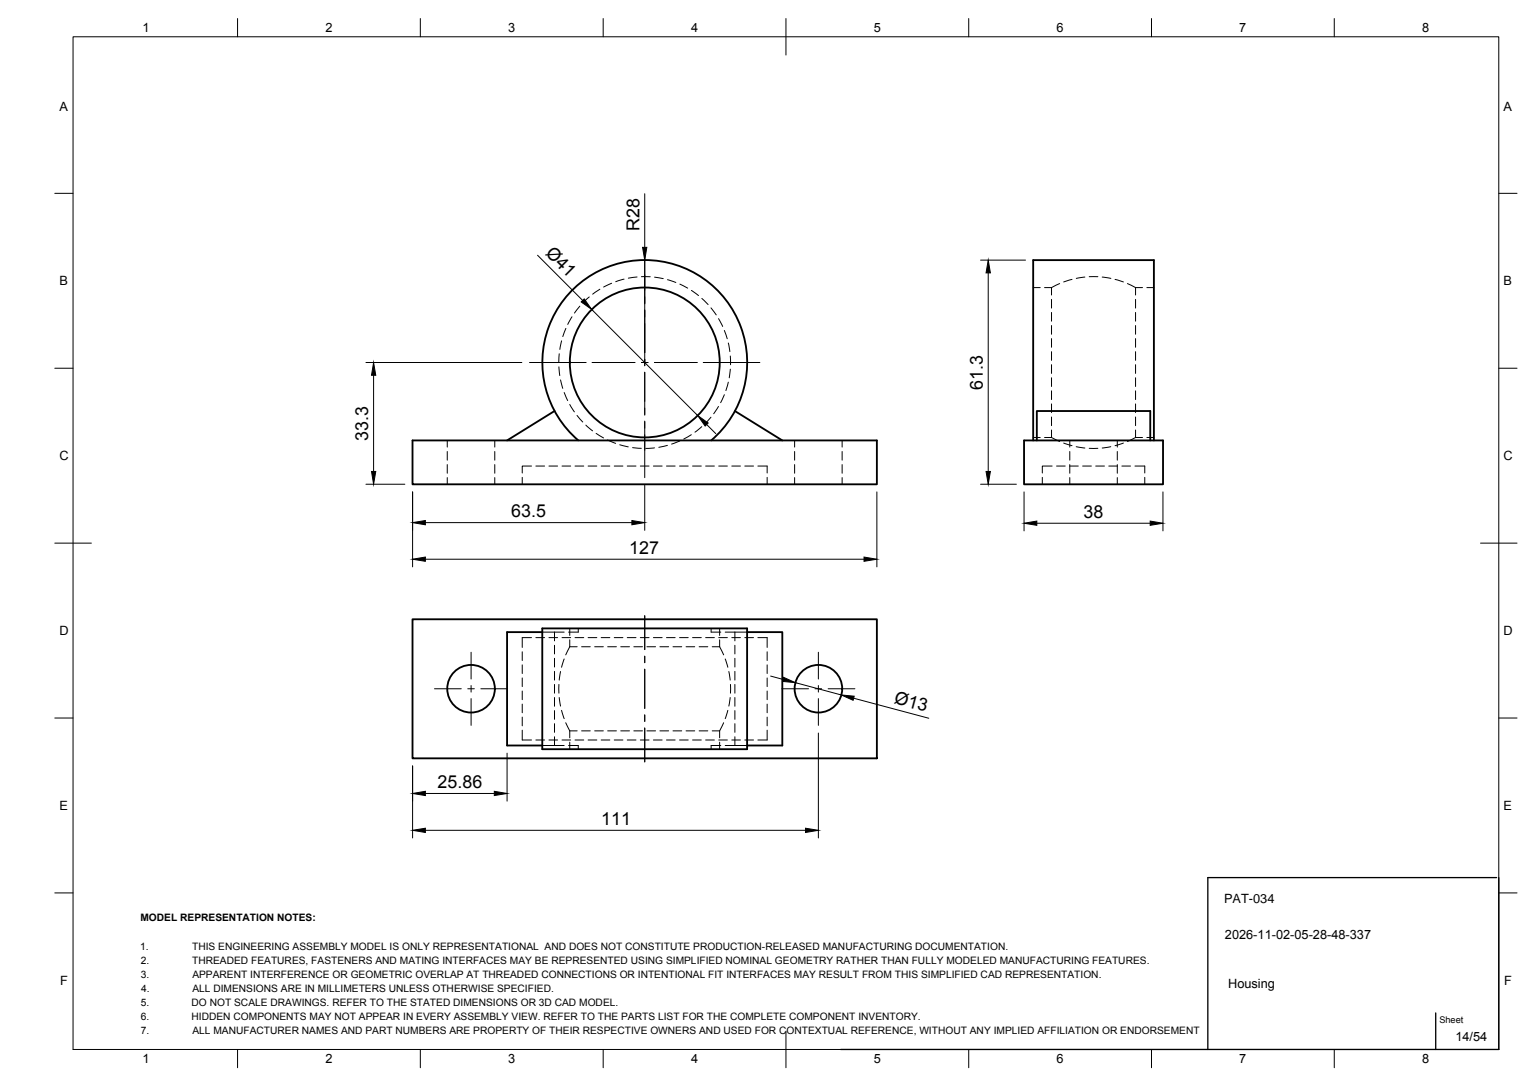
ISO-10303-21;
HEADER;
/* Generated by software containing ST-Developer
 * from STEP Tools, Inc. (www.steptools.com) 
 */

FILE_DESCRIPTION(
/* description */ ('Fatigue rig crank-slider'),
/* implementation_level */ '2;1');

FILE_NAME(
/* name */ 'Housing.step',
/* time_stamp */ '2026-10-28T03:24:50-07:00',
/* author */ (''),
/* organization */ (''),
/* preprocessor_version */ 'ST-DEVELOPER v20.2',
/* originating_system */ 'Autodesk Translation Framework v15.17.0.0',
/* authorisation */ '');

FILE_SCHEMA (('AUTOMOTIVE_DESIGN { 1 0 10303 214 3 1 1 }'));
ENDSEC;

DATA;
#10=MECHANICAL_DESIGN_GEOMETRIC_PRESENTATION_REPRESENTATION('',(#597),#16911);
#469=SPHERICAL_SURFACE('',#9733,2.35);
#497=SHAPE_REPRESENTATION_RELATIONSHIP('SRR','None',#17137,#547);
#547=ADVANCED_BREP_SHAPE_REPRESENTATION('',(#656),#16866);
#597=STYLED_ITEM('',(#17466),#656);
#656=MANIFOLD_SOLID_BREP('Body1',#8888);
#776=FACE_BOUND('',#1935,.T.);
#777=FACE_BOUND('',#1936,.T.);
#778=FACE_BOUND('',#1944,.T.);
#779=FACE_BOUND('',#1945,.T.);
#780=FACE_BOUND('',#1946,.T.);
#781=FACE_BOUND('',#1949,.T.);
#782=FACE_BOUND('',#1951,.T.);
#783=FACE_BOUND('',#1964,.T.);
#784=FACE_BOUND('',#1965,.T.);
#785=FACE_BOUND('',#1966,.T.);
#961=PLANE('',#9735);
#962=PLANE('',#9737);
#963=PLANE('',#9739);
#964=PLANE('',#9741);
#965=PLANE('',#9742);
#966=PLANE('',#9744);
#967=PLANE('',#9745);
#968=PLANE('',#9751);
#969=PLANE('',#9752);
#970=PLANE('',#9753);
#971=PLANE('',#9754);
#972=PLANE('',#9755);
#973=PLANE('',#9756);
#974=PLANE('',#9757);
#975=PLANE('',#9762);
#976=PLANE('',#9763);
#977=PLANE('',#9764);
#978=PLANE('',#9765);
#979=PLANE('',#9766);
#1333=FACE_OUTER_BOUND('',#1932,.T.);
#1334=FACE_OUTER_BOUND('',#1933,.T.);
#1335=FACE_OUTER_BOUND('',#1934,.T.);
#1336=FACE_OUTER_BOUND('',#1937,.T.);
#1337=FACE_OUTER_BOUND('',#1938,.T.);
#1338=FACE_OUTER_BOUND('',#1939,.T.);
#1339=FACE_OUTER_BOUND('',#1940,.T.);
#1340=FACE_OUTER_BOUND('',#1941,.T.);
#1341=FACE_OUTER_BOUND('',#1942,.T.);
#1342=FACE_OUTER_BOUND('',#1943,.T.);
#1343=FACE_OUTER_BOUND('',#1947,.T.);
#1344=FACE_OUTER_BOUND('',#1948,.T.);
#1345=FACE_OUTER_BOUND('',#1950,.T.);
#1346=FACE_OUTER_BOUND('',#1952,.T.);
#1347=FACE_OUTER_BOUND('',#1953,.T.);
#1348=FACE_OUTER_BOUND('',#1954,.T.);
#1349=FACE_OUTER_BOUND('',#1955,.T.);
#1350=FACE_OUTER_BOUND('',#1956,.T.);
#1351=FACE_OUTER_BOUND('',#1957,.T.);
#1352=FACE_OUTER_BOUND('',#1958,.T.);
#1353=FACE_OUTER_BOUND('',#1959,.T.);
#1354=FACE_OUTER_BOUND('',#1960,.T.);
#1355=FACE_OUTER_BOUND('',#1961,.T.);
#1356=FACE_OUTER_BOUND('',#1962,.T.);
#1357=FACE_OUTER_BOUND('',#1963,.T.);
#1932=EDGE_LOOP('',(#6452,#6453,#6454,#6455));
#1933=EDGE_LOOP('',(#6456,#6457,#6458,#6459));
#1934=EDGE_LOOP('',(#6460,#6461));
#1935=EDGE_LOOP('',(#6462));
#1936=EDGE_LOOP('',(#6463));
#1937=EDGE_LOOP('',(#6464,#6465,#6466));
#1938=EDGE_LOOP('',(#6467,#6468,#6469));
#1939=EDGE_LOOP('',(#6470,#6471,#6472));
#1940=EDGE_LOOP('',(#6473,#6474,#6475,#6476));
#1941=EDGE_LOOP('',(#6477,#6478,#6479));
#1942=EDGE_LOOP('',(#6480,#6481,#6482,#6483));
#1943=EDGE_LOOP('',(#6484,#6485,#6486,#6487));
#1944=EDGE_LOOP('',(#6488));
#1945=EDGE_LOOP('',(#6489));
#1946=EDGE_LOOP('',(#6490,#6491,#6492,#6493,#6494,#6495,#6496,#6497,#6498,
#6499,#6500,#6501));
#1947=EDGE_LOOP('',(#6502,#6503,#6504,#6505,#6506,#6507,#6508,#6509,#6510,
#6511,#6512,#6513));
#1948=EDGE_LOOP('',(#6514,#6515));
#1949=EDGE_LOOP('',(#6516));
#1950=EDGE_LOOP('',(#6517,#6518));
#1951=EDGE_LOOP('',(#6519));
#1952=EDGE_LOOP('',(#6520,#6521,#6522,#6523));
#1953=EDGE_LOOP('',(#6524,#6525,#6526,#6527));
#1954=EDGE_LOOP('',(#6528,#6529,#6530,#6531));
#1955=EDGE_LOOP('',(#6532,#6533,#6534,#6535));
#1956=EDGE_LOOP('',(#6536,#6537,#6538,#6539));
#1957=EDGE_LOOP('',(#6540,#6541,#6542,#6543));
#1958=EDGE_LOOP('',(#6544,#6545,#6546,#6547));
#1959=EDGE_LOOP('',(#6548,#6549,#6550,#6551));
#1960=EDGE_LOOP('',(#6552,#6553,#6554,#6555));
#1961=EDGE_LOOP('',(#6556,#6557,#6558,#6559));
#1962=EDGE_LOOP('',(#6560,#6561,#6562,#6563));
#1963=EDGE_LOOP('',(#6564,#6565,#6566,#6567));
#1964=EDGE_LOOP('',(#6568,#6569,#6570,#6571));
#1965=EDGE_LOOP('',(#6572));
#1966=EDGE_LOOP('',(#6573));
#2584=LINE('',#13872,#3230);
#2585=LINE('',#13878,#3231);
#2586=LINE('',#13887,#3232);
#2587=LINE('',#13889,#3233);
#2588=LINE('',#13894,#3234);
#2589=LINE('',#13897,#3235);
#2590=LINE('',#13901,#3236);
#2591=LINE('',#13904,#3237);
#2592=LINE('',#13906,#3238);
#2593=LINE('',#13907,#3239);
#2594=LINE('',#13911,#3240);
#2595=LINE('',#13913,#3241);
#2596=LINE('',#13916,#3242);
#2597=LINE('',#13917,#3243);
#2598=LINE('',#13921,#3244);
#2599=LINE('',#13923,#3245);
#2600=LINE('',#13925,#3246);
#2601=LINE('',#13926,#3247);
#2602=LINE('',#13932,#3248);
#2603=LINE('',#13934,#3249);
#2604=LINE('',#13935,#3250);
#2605=LINE('',#13937,#3251);
#2606=LINE('',#13939,#3252);
#2607=LINE('',#13940,#3253);
#2608=LINE('',#13949,#3254);
#2609=LINE('',#13951,#3255);
#2610=LINE('',#13953,#3256);
#2611=LINE('',#13954,#3257);
#2612=LINE('',#13957,#3258);
#2613=LINE('',#13959,#3259);
#2614=LINE('',#13960,#3260);
#2615=LINE('',#13963,#3261);
#2616=LINE('',#13965,#3262);
#2617=LINE('',#13966,#3263);
#2618=LINE('',#13968,#3264);
#2619=LINE('',#13969,#3265);
#2620=LINE('',#13974,#3266);
#2621=LINE('',#13978,#3267);
#2622=LINE('',#13982,#3268);
#2623=LINE('',#13983,#3269);
#2624=LINE('',#13984,#3270);
#2625=LINE('',#13987,#3271);
#2626=LINE('',#13988,#3272);
#2627=LINE('',#13991,#3273);
#2628=LINE('',#13992,#3274);
#2629=LINE('',#13994,#3275);
#3230=VECTOR('',#11162,2.05);
#3231=VECTOR('',#11169,2.05);
#3232=VECTOR('',#11178,1.);
#3233=VECTOR('',#11179,1.);
#3234=VECTOR('',#11184,1.);
#3235=VECTOR('',#11187,1.);
#3236=VECTOR('',#11190,1.);
#3237=VECTOR('',#11193,1.);
#3238=VECTOR('',#11196,1.);
#3239=VECTOR('',#11197,1.);
#3240=VECTOR('',#11200,1.);
#3241=VECTOR('',#11201,1.);
#3242=VECTOR('',#11206,1.);
#3243=VECTOR('',#11207,1.);
#3244=VECTOR('',#11210,1.);
#3245=VECTOR('',#11211,1.);
#3246=VECTOR('',#11212,1.);
#3247=VECTOR('',#11213,1.);
#3248=VECTOR('',#11218,1.);
#3249=VECTOR('',#11219,1.);
#3250=VECTOR('',#11220,1.);
#3251=VECTOR('',#11221,1.);
#3252=VECTOR('',#11222,1.);
#3253=VECTOR('',#11223,1.);
#3254=VECTOR('',#11236,1.);
#3255=VECTOR('',#11237,1.);
#3256=VECTOR('',#11238,1.);
#3257=VECTOR('',#11239,1.);
#3258=VECTOR('',#11242,1.);
#3259=VECTOR('',#11243,1.);
#3260=VECTOR('',#11244,1.);
#3261=VECTOR('',#11247,1.);
#3262=VECTOR('',#11248,1.);
#3263=VECTOR('',#11249,1.);
#3264=VECTOR('',#11252,1.);
#3265=VECTOR('',#11253,1.);
#3266=VECTOR('',#11260,0.65);
#3267=VECTOR('',#11265,0.65);
#3268=VECTOR('',#11268,1.);
#3269=VECTOR('',#11269,1.);
#3270=VECTOR('',#11270,1.);
#3271=VECTOR('',#11273,1.);
#3272=VECTOR('',#11274,1.);
#3273=VECTOR('',#11277,1.);
#3274=VECTOR('',#11278,1.);
#3275=VECTOR('',#11281,1.);
#3856=CIRCLE('',#9728,2.05);
#3857=CIRCLE('',#9729,2.05);
#3858=CIRCLE('',#9731,2.05);
#3859=CIRCLE('',#9732,2.05);
#3860=CIRCLE('',#9734,2.35);
#3861=CIRCLE('',#9736,2.8);
#3862=CIRCLE('',#9738,2.8);
#3863=CIRCLE('',#9740,2.8);
#3864=CIRCLE('',#9743,2.8);
#3865=CIRCLE('',#9746,0.65);
#3866=CIRCLE('',#9747,0.65);
#3867=CIRCLE('',#9749,2.8);
#3868=CIRCLE('',#9750,2.8);
#3869=CIRCLE('',#9759,0.65);
#3870=CIRCLE('',#9761,0.65);
#4304=VERTEX_POINT('',#13869);
#4305=VERTEX_POINT('',#13871);
#4306=VERTEX_POINT('',#13875);
#4307=VERTEX_POINT('',#13877);
#4308=VERTEX_POINT('',#13881);
#4309=VERTEX_POINT('',#13882);
#4310=VERTEX_POINT('',#13885);
#4311=VERTEX_POINT('',#13886);
#4312=VERTEX_POINT('',#13888);
#4313=VERTEX_POINT('',#13892);
#4314=VERTEX_POINT('',#13893);
#4315=VERTEX_POINT('',#13895);
#4316=VERTEX_POINT('',#13899);
#4317=VERTEX_POINT('',#13900);
#4318=VERTEX_POINT('',#13902);
#4319=VERTEX_POINT('',#13909);
#4320=VERTEX_POINT('',#13910);
#4321=VERTEX_POINT('',#13912);
#4322=VERTEX_POINT('',#13919);
#4323=VERTEX_POINT('',#13920);
#4324=VERTEX_POINT('',#13922);
#4325=VERTEX_POINT('',#13924);
#4326=VERTEX_POINT('',#13927);
#4327=VERTEX_POINT('',#13929);
#4328=VERTEX_POINT('',#13931);
#4329=VERTEX_POINT('',#13933);
#4330=VERTEX_POINT('',#13936);
#4331=VERTEX_POINT('',#13938);
#4332=VERTEX_POINT('',#13947);
#4333=VERTEX_POINT('',#13948);
#4334=VERTEX_POINT('',#13950);
#4335=VERTEX_POINT('',#13952);
#4336=VERTEX_POINT('',#13956);
#4337=VERTEX_POINT('',#13958);
#4338=VERTEX_POINT('',#13962);
#4339=VERTEX_POINT('',#13964);
#4340=VERTEX_POINT('',#13972);
#4341=VERTEX_POINT('',#13976);
#4342=VERTEX_POINT('',#13980);
#4343=VERTEX_POINT('',#13981);
#4344=VERTEX_POINT('',#13986);
#4345=VERTEX_POINT('',#13990);
#5124=EDGE_CURVE('',#4304,#4304,#3856,.T.);
#5125=EDGE_CURVE('',#4304,#4305,#2584,.T.);
#5126=EDGE_CURVE('',#4305,#4305,#3857,.T.);
#5127=EDGE_CURVE('',#4306,#4306,#3858,.T.);
#5128=EDGE_CURVE('',#4306,#4307,#2585,.T.);
#5129=EDGE_CURVE('',#4307,#4307,#3859,.T.);
#5130=EDGE_CURVE('',#4308,#4309,#3860,.T.);
#5131=EDGE_CURVE('',#4310,#4311,#2586,.T.);
#5132=EDGE_CURVE('',#4310,#4312,#2587,.T.);
#5133=EDGE_CURVE('',#4311,#4312,#3861,.T.);
#5134=EDGE_CURVE('',#4313,#4314,#2588,.T.);
#5135=EDGE_CURVE('',#4315,#4313,#3862,.T.);
#5136=EDGE_CURVE('',#4315,#4314,#2589,.T.);
#5137=EDGE_CURVE('',#4316,#4317,#2590,.T.);
#5138=EDGE_CURVE('',#4318,#4316,#3863,.T.);
#5139=EDGE_CURVE('',#4318,#4317,#2591,.T.);
#5140=EDGE_CURVE('',#4317,#4310,#2592,.T.);
#5141=EDGE_CURVE('',#4312,#4318,#2593,.T.);
#5142=EDGE_CURVE('',#4319,#4320,#2594,.T.);
#5143=EDGE_CURVE('',#4319,#4321,#2595,.T.);
#5144=EDGE_CURVE('',#4320,#4321,#3864,.T.);
#5145=EDGE_CURVE('',#4314,#4319,#2596,.T.);
#5146=EDGE_CURVE('',#4321,#4315,#2597,.T.);
#5147=EDGE_CURVE('',#4322,#4323,#2598,.T.);
#5148=EDGE_CURVE('',#4323,#4324,#2599,.T.);
#5149=EDGE_CURVE('',#4324,#4325,#2600,.T.);
#5150=EDGE_CURVE('',#4325,#4322,#2601,.T.);
#5151=EDGE_CURVE('',#4326,#4326,#3865,.T.);
#5152=EDGE_CURVE('',#4327,#4327,#3866,.T.);
#5153=EDGE_CURVE('',#4320,#4328,#2602,.T.);
#5154=EDGE_CURVE('',#4328,#4329,#2603,.T.);
#5155=EDGE_CURVE('',#4329,#4316,#2604,.T.);
#5156=EDGE_CURVE('',#4311,#4330,#2605,.T.);
#5157=EDGE_CURVE('',#4330,#4331,#2606,.T.);
#5158=EDGE_CURVE('',#4331,#4313,#2607,.T.);
#5159=EDGE_CURVE('',#4330,#4331,#3867,.T.);
#5160=EDGE_CURVE('',#4328,#4329,#3868,.T.);
#5161=EDGE_CURVE('',#4332,#4333,#2608,.T.);
#5162=EDGE_CURVE('',#4332,#4334,#2609,.T.);
#5163=EDGE_CURVE('',#4334,#4335,#2610,.T.);
#5164=EDGE_CURVE('',#4333,#4335,#2611,.T.);
#5165=EDGE_CURVE('',#4336,#4332,#2612,.T.);
#5166=EDGE_CURVE('',#4336,#4337,#2613,.T.);
#5167=EDGE_CURVE('',#4337,#4334,#2614,.T.);
#5168=EDGE_CURVE('',#4338,#4336,#2615,.T.);
#5169=EDGE_CURVE('',#4338,#4339,#2616,.T.);
#5170=EDGE_CURVE('',#4339,#4337,#2617,.T.);
#5171=EDGE_CURVE('',#4333,#4338,#2618,.T.);
#5172=EDGE_CURVE('',#4335,#4339,#2619,.T.);
#5173=EDGE_CURVE('',#4340,#4340,#3869,.T.);
#5174=EDGE_CURVE('',#4340,#4327,#2620,.T.);
#5175=EDGE_CURVE('',#4341,#4341,#3870,.T.);
#5176=EDGE_CURVE('',#4341,#4326,#2621,.T.);
#5177=EDGE_CURVE('',#4342,#4343,#2622,.T.);
#5178=EDGE_CURVE('',#4343,#4322,#2623,.T.);
#5179=EDGE_CURVE('',#4342,#4325,#2624,.T.);
#5180=EDGE_CURVE('',#4344,#4342,#2625,.T.);
#5181=EDGE_CURVE('',#4344,#4324,#2626,.T.);
#5182=EDGE_CURVE('',#4345,#4344,#2627,.T.);
#5183=EDGE_CURVE('',#4345,#4323,#2628,.T.);
#5184=EDGE_CURVE('',#4343,#4345,#2629,.T.);
#6452=ORIENTED_EDGE('',*,*,#5124,.F.);
#6453=ORIENTED_EDGE('',*,*,#5125,.T.);
#6454=ORIENTED_EDGE('',*,*,#5126,.F.);
#6455=ORIENTED_EDGE('',*,*,#5125,.F.);
#6456=ORIENTED_EDGE('',*,*,#5127,.F.);
#6457=ORIENTED_EDGE('',*,*,#5128,.T.);
#6458=ORIENTED_EDGE('',*,*,#5129,.F.);
#6459=ORIENTED_EDGE('',*,*,#5128,.F.);
#6460=ORIENTED_EDGE('',*,*,#5130,.T.);
#6461=ORIENTED_EDGE('',*,*,#5130,.F.);
#6462=ORIENTED_EDGE('',*,*,#5127,.T.);
#6463=ORIENTED_EDGE('',*,*,#5126,.T.);
#6464=ORIENTED_EDGE('',*,*,#5131,.F.);
#6465=ORIENTED_EDGE('',*,*,#5132,.T.);
#6466=ORIENTED_EDGE('',*,*,#5133,.F.);
#6467=ORIENTED_EDGE('',*,*,#5134,.F.);
#6468=ORIENTED_EDGE('',*,*,#5135,.F.);
#6469=ORIENTED_EDGE('',*,*,#5136,.T.);
#6470=ORIENTED_EDGE('',*,*,#5137,.F.);
#6471=ORIENTED_EDGE('',*,*,#5138,.F.);
#6472=ORIENTED_EDGE('',*,*,#5139,.T.);
#6473=ORIENTED_EDGE('',*,*,#5140,.F.);
#6474=ORIENTED_EDGE('',*,*,#5139,.F.);
#6475=ORIENTED_EDGE('',*,*,#5141,.F.);
#6476=ORIENTED_EDGE('',*,*,#5132,.F.);
#6477=ORIENTED_EDGE('',*,*,#5142,.F.);
#6478=ORIENTED_EDGE('',*,*,#5143,.T.);
#6479=ORIENTED_EDGE('',*,*,#5144,.F.);
#6480=ORIENTED_EDGE('',*,*,#5145,.F.);
#6481=ORIENTED_EDGE('',*,*,#5136,.F.);
#6482=ORIENTED_EDGE('',*,*,#5146,.F.);
#6483=ORIENTED_EDGE('',*,*,#5143,.F.);
#6484=ORIENTED_EDGE('',*,*,#5147,.T.);
#6485=ORIENTED_EDGE('',*,*,#5148,.T.);
#6486=ORIENTED_EDGE('',*,*,#5149,.T.);
#6487=ORIENTED_EDGE('',*,*,#5150,.T.);
#6488=ORIENTED_EDGE('',*,*,#5151,.T.);
#6489=ORIENTED_EDGE('',*,*,#5152,.T.);
#6490=ORIENTED_EDGE('',*,*,#5134,.T.);
#6491=ORIENTED_EDGE('',*,*,#5145,.T.);
#6492=ORIENTED_EDGE('',*,*,#5142,.T.);
#6493=ORIENTED_EDGE('',*,*,#5153,.T.);
#6494=ORIENTED_EDGE('',*,*,#5154,.T.);
#6495=ORIENTED_EDGE('',*,*,#5155,.T.);
#6496=ORIENTED_EDGE('',*,*,#5137,.T.);
#6497=ORIENTED_EDGE('',*,*,#5140,.T.);
#6498=ORIENTED_EDGE('',*,*,#5131,.T.);
#6499=ORIENTED_EDGE('',*,*,#5156,.T.);
#6500=ORIENTED_EDGE('',*,*,#5157,.T.);
#6501=ORIENTED_EDGE('',*,*,#5158,.T.);
#6502=ORIENTED_EDGE('',*,*,#5135,.T.);
#6503=ORIENTED_EDGE('',*,*,#5158,.F.);
#6504=ORIENTED_EDGE('',*,*,#5159,.F.);
#6505=ORIENTED_EDGE('',*,*,#5156,.F.);
#6506=ORIENTED_EDGE('',*,*,#5133,.T.);
#6507=ORIENTED_EDGE('',*,*,#5141,.T.);
#6508=ORIENTED_EDGE('',*,*,#5138,.T.);
#6509=ORIENTED_EDGE('',*,*,#5155,.F.);
#6510=ORIENTED_EDGE('',*,*,#5160,.F.);
#6511=ORIENTED_EDGE('',*,*,#5153,.F.);
#6512=ORIENTED_EDGE('',*,*,#5144,.T.);
#6513=ORIENTED_EDGE('',*,*,#5146,.T.);
#6514=ORIENTED_EDGE('',*,*,#5154,.F.);
#6515=ORIENTED_EDGE('',*,*,#5160,.T.);
#6516=ORIENTED_EDGE('',*,*,#5124,.T.);
#6517=ORIENTED_EDGE('',*,*,#5157,.F.);
#6518=ORIENTED_EDGE('',*,*,#5159,.T.);
#6519=ORIENTED_EDGE('',*,*,#5129,.T.);
#6520=ORIENTED_EDGE('',*,*,#5161,.F.);
#6521=ORIENTED_EDGE('',*,*,#5162,.T.);
#6522=ORIENTED_EDGE('',*,*,#5163,.T.);
#6523=ORIENTED_EDGE('',*,*,#5164,.F.);
#6524=ORIENTED_EDGE('',*,*,#5165,.F.);
#6525=ORIENTED_EDGE('',*,*,#5166,.T.);
#6526=ORIENTED_EDGE('',*,*,#5167,.T.);
#6527=ORIENTED_EDGE('',*,*,#5162,.F.);
#6528=ORIENTED_EDGE('',*,*,#5168,.F.);
#6529=ORIENTED_EDGE('',*,*,#5169,.T.);
#6530=ORIENTED_EDGE('',*,*,#5170,.T.);
#6531=ORIENTED_EDGE('',*,*,#5166,.F.);
#6532=ORIENTED_EDGE('',*,*,#5171,.F.);
#6533=ORIENTED_EDGE('',*,*,#5164,.T.);
#6534=ORIENTED_EDGE('',*,*,#5172,.T.);
#6535=ORIENTED_EDGE('',*,*,#5169,.F.);
#6536=ORIENTED_EDGE('',*,*,#5172,.F.);
#6537=ORIENTED_EDGE('',*,*,#5163,.F.);
#6538=ORIENTED_EDGE('',*,*,#5167,.F.);
#6539=ORIENTED_EDGE('',*,*,#5170,.F.);
#6540=ORIENTED_EDGE('',*,*,#5173,.F.);
#6541=ORIENTED_EDGE('',*,*,#5174,.T.);
#6542=ORIENTED_EDGE('',*,*,#5152,.F.);
#6543=ORIENTED_EDGE('',*,*,#5174,.F.);
#6544=ORIENTED_EDGE('',*,*,#5175,.F.);
#6545=ORIENTED_EDGE('',*,*,#5176,.T.);
#6546=ORIENTED_EDGE('',*,*,#5151,.F.);
#6547=ORIENTED_EDGE('',*,*,#5176,.F.);
#6548=ORIENTED_EDGE('',*,*,#5177,.T.);
#6549=ORIENTED_EDGE('',*,*,#5178,.T.);
#6550=ORIENTED_EDGE('',*,*,#5150,.F.);
#6551=ORIENTED_EDGE('',*,*,#5179,.F.);
#6552=ORIENTED_EDGE('',*,*,#5180,.T.);
#6553=ORIENTED_EDGE('',*,*,#5179,.T.);
#6554=ORIENTED_EDGE('',*,*,#5149,.F.);
#6555=ORIENTED_EDGE('',*,*,#5181,.F.);
#6556=ORIENTED_EDGE('',*,*,#5182,.T.);
#6557=ORIENTED_EDGE('',*,*,#5181,.T.);
#6558=ORIENTED_EDGE('',*,*,#5148,.F.);
#6559=ORIENTED_EDGE('',*,*,#5183,.F.);
#6560=ORIENTED_EDGE('',*,*,#5184,.T.);
#6561=ORIENTED_EDGE('',*,*,#5183,.T.);
#6562=ORIENTED_EDGE('',*,*,#5147,.F.);
#6563=ORIENTED_EDGE('',*,*,#5178,.F.);
#6564=ORIENTED_EDGE('',*,*,#5184,.F.);
#6565=ORIENTED_EDGE('',*,*,#5177,.F.);
#6566=ORIENTED_EDGE('',*,*,#5180,.F.);
#6567=ORIENTED_EDGE('',*,*,#5182,.F.);
#6568=ORIENTED_EDGE('',*,*,#5161,.T.);
#6569=ORIENTED_EDGE('',*,*,#5171,.T.);
#6570=ORIENTED_EDGE('',*,*,#5168,.T.);
#6571=ORIENTED_EDGE('',*,*,#5165,.T.);
#6572=ORIENTED_EDGE('',*,*,#5173,.T.);
#6573=ORIENTED_EDGE('',*,*,#5175,.T.);
#8248=CYLINDRICAL_SURFACE('',#9727,2.05);
#8249=CYLINDRICAL_SURFACE('',#9730,2.05);
#8250=CYLINDRICAL_SURFACE('',#9748,2.8);
#8251=CYLINDRICAL_SURFACE('',#9758,0.65);
#8252=CYLINDRICAL_SURFACE('',#9760,0.65);
#8471=ADVANCED_FACE('',(#1333),#8248,.F.);
#8472=ADVANCED_FACE('',(#1334),#8249,.F.);
#8473=ADVANCED_FACE('',(#1335,#776,#777),#469,.F.);
#8474=ADVANCED_FACE('',(#1336),#961,.T.);
#8475=ADVANCED_FACE('',(#1337),#962,.T.);
#8476=ADVANCED_FACE('',(#1338),#963,.T.);
#8477=ADVANCED_FACE('',(#1339),#964,.T.);
#8478=ADVANCED_FACE('',(#1340),#965,.T.);
#8479=ADVANCED_FACE('',(#1341),#966,.T.);
#8480=ADVANCED_FACE('',(#1342,#778,#779,#780),#967,.T.);
#8481=ADVANCED_FACE('',(#1343),#8250,.T.);
#8482=ADVANCED_FACE('',(#1344,#781),#968,.F.);
#8483=ADVANCED_FACE('',(#1345,#782),#969,.T.);
#8484=ADVANCED_FACE('',(#1346),#970,.F.);
#8485=ADVANCED_FACE('',(#1347),#971,.F.);
#8486=ADVANCED_FACE('',(#1348),#972,.F.);
#8487=ADVANCED_FACE('',(#1349),#973,.F.);
#8488=ADVANCED_FACE('',(#1350),#974,.F.);
#8489=ADVANCED_FACE('',(#1351),#8251,.F.);
#8490=ADVANCED_FACE('',(#1352),#8252,.F.);
#8491=ADVANCED_FACE('',(#1353),#975,.T.);
#8492=ADVANCED_FACE('',(#1354),#976,.T.);
#8493=ADVANCED_FACE('',(#1355),#977,.T.);
#8494=ADVANCED_FACE('',(#1356),#978,.T.);
#8495=ADVANCED_FACE('',(#1357,#783,#784,#785),#979,.F.);
#8888=CLOSED_SHELL('',(#8471,#8472,#8473,#8474,#8475,#8476,#8477,#8478,
#8479,#8480,#8481,#8482,#8483,#8484,#8485,#8486,#8487,#8488,#8489,#8490,
#8491,#8492,#8493,#8494,#8495));
#9726=AXIS2_PLACEMENT_3D('',#13867,#11156,#11157);
#9727=AXIS2_PLACEMENT_3D('',#13868,#11158,#11159);
#9728=AXIS2_PLACEMENT_3D('',#13870,#11160,#11161);
#9729=AXIS2_PLACEMENT_3D('',#13873,#11163,#11164);
#9730=AXIS2_PLACEMENT_3D('',#13874,#11165,#11166);
#9731=AXIS2_PLACEMENT_3D('',#13876,#11167,#11168);
#9732=AXIS2_PLACEMENT_3D('',#13879,#11170,#11171);
#9733=AXIS2_PLACEMENT_3D('',#13880,#11172,#11173);
#9734=AXIS2_PLACEMENT_3D('',#13883,#11174,#11175);
#9735=AXIS2_PLACEMENT_3D('',#13884,#11176,#11177);
#9736=AXIS2_PLACEMENT_3D('',#13890,#11180,#11181);
#9737=AXIS2_PLACEMENT_3D('',#13891,#11182,#11183);
#9738=AXIS2_PLACEMENT_3D('',#13896,#11185,#11186);
#9739=AXIS2_PLACEMENT_3D('',#13898,#11188,#11189);
#9740=AXIS2_PLACEMENT_3D('',#13903,#11191,#11192);
#9741=AXIS2_PLACEMENT_3D('',#13905,#11194,#11195);
#9742=AXIS2_PLACEMENT_3D('',#13908,#11198,#11199);
#9743=AXIS2_PLACEMENT_3D('',#13914,#11202,#11203);
#9744=AXIS2_PLACEMENT_3D('',#13915,#11204,#11205);
#9745=AXIS2_PLACEMENT_3D('',#13918,#11208,#11209);
#9746=AXIS2_PLACEMENT_3D('',#13928,#11214,#11215);
#9747=AXIS2_PLACEMENT_3D('',#13930,#11216,#11217);
#9748=AXIS2_PLACEMENT_3D('',#13941,#11224,#11225);
#9749=AXIS2_PLACEMENT_3D('',#13942,#11226,#11227);
#9750=AXIS2_PLACEMENT_3D('',#13943,#11228,#11229);
#9751=AXIS2_PLACEMENT_3D('',#13944,#11230,#11231);
#9752=AXIS2_PLACEMENT_3D('',#13945,#11232,#11233);
#9753=AXIS2_PLACEMENT_3D('',#13946,#11234,#11235);
#9754=AXIS2_PLACEMENT_3D('',#13955,#11240,#11241);
#9755=AXIS2_PLACEMENT_3D('',#13961,#11245,#11246);
#9756=AXIS2_PLACEMENT_3D('',#13967,#11250,#11251);
#9757=AXIS2_PLACEMENT_3D('',#13970,#11254,#11255);
#9758=AXIS2_PLACEMENT_3D('',#13971,#11256,#11257);
#9759=AXIS2_PLACEMENT_3D('',#13973,#11258,#11259);
#9760=AXIS2_PLACEMENT_3D('',#13975,#11261,#11262);
#9761=AXIS2_PLACEMENT_3D('',#13977,#11263,#11264);
#9762=AXIS2_PLACEMENT_3D('',#13979,#11266,#11267);
#9763=AXIS2_PLACEMENT_3D('',#13985,#11271,#11272);
#9764=AXIS2_PLACEMENT_3D('',#13989,#11275,#11276);
#9765=AXIS2_PLACEMENT_3D('',#13993,#11279,#11280);
#9766=AXIS2_PLACEMENT_3D('',#13995,#11282,#11283);
#11156=DIRECTION('axis',(0.,0.,1.));
#11157=DIRECTION('refdir',(1.,0.,0.));
#11158=DIRECTION('center_axis',(0.,1.,0.));
#11159=DIRECTION('ref_axis',(1.,0.,0.));
#11160=DIRECTION('center_axis',(0.,1.,0.));
#11161=DIRECTION('ref_axis',(1.,0.,0.));
#11162=DIRECTION('',(0.,1.,0.));
#11163=DIRECTION('center_axis',(0.,-1.,0.));
#11164=DIRECTION('ref_axis',(1.,0.,0.));
#11165=DIRECTION('center_axis',(0.,1.,0.));
#11166=DIRECTION('ref_axis',(1.,0.,0.));
#11167=DIRECTION('center_axis',(0.,1.,0.));
#11168=DIRECTION('ref_axis',(1.,0.,0.));
#11169=DIRECTION('',(0.,1.,0.));
#11170=DIRECTION('center_axis',(0.,-1.,0.));
#11171=DIRECTION('ref_axis',(1.,0.,0.));
#11172=DIRECTION('center_axis',(6.12323399573677E-17,0.,1.));
#11173=DIRECTION('ref_axis',(1.,0.,0.));
#11174=DIRECTION('center_axis',(-1.22464679914735E-16,1.,0.));
#11175=DIRECTION('ref_axis',(-1.,-1.22464679914735E-16,0.));
#11176=DIRECTION('center_axis',(0.,1.,0.));
#11177=DIRECTION('ref_axis',(0.,0.,1.));
#11178=DIRECTION('',(1.,0.,0.));
#11179=DIRECTION('',(0.850265146687862,0.,0.526354614616295));
#11180=DIRECTION('center_axis',(0.,1.,0.));
#11181=DIRECTION('ref_axis',(1.,0.,0.));
#11182=DIRECTION('center_axis',(0.,1.,0.));
#11183=DIRECTION('ref_axis',(0.,0.,1.));
#11184=DIRECTION('',(1.,0.,0.));
#11185=DIRECTION('center_axis',(0.,1.,0.));
#11186=DIRECTION('ref_axis',(1.,0.,0.));
#11187=DIRECTION('',(0.850265146687862,0.,-0.526354614616295));
#11188=DIRECTION('center_axis',(0.,-1.,0.));
#11189=DIRECTION('ref_axis',(0.,0.,-1.));
#11190=DIRECTION('',(-1.,0.,0.));
#11191=DIRECTION('center_axis',(0.,-1.,0.));
#11192=DIRECTION('ref_axis',(1.,0.,0.));
#11193=DIRECTION('',(-0.850265146687862,0.,-0.526354614616295));
#11194=DIRECTION('center_axis',(-0.526354614616295,0.,0.850265146687862));
#11195=DIRECTION('ref_axis',(0.850265146687862,0.,0.526354614616295));
#11196=DIRECTION('',(0.,1.,0.));
#11197=DIRECTION('',(0.,-1.,0.));
#11198=DIRECTION('center_axis',(0.,-1.,0.));
#11199=DIRECTION('ref_axis',(0.,0.,-1.));
#11200=DIRECTION('',(-1.,0.,0.));
#11201=DIRECTION('',(-0.850265146687862,0.,0.526354614616295));
#11202=DIRECTION('center_axis',(0.,-1.,0.));
#11203=DIRECTION('ref_axis',(1.,0.,0.));
#11204=DIRECTION('center_axis',(0.526354614616295,0.,0.850265146687862));
#11205=DIRECTION('ref_axis',(0.850265146687862,0.,-0.526354614616295));
#11206=DIRECTION('',(0.,-1.,0.));
#11207=DIRECTION('',(0.,1.,0.));
#11208=DIRECTION('center_axis',(0.,0.,1.));
#11209=DIRECTION('ref_axis',(1.,0.,0.));
#11210=DIRECTION('',(0.,-1.,0.));
#11211=DIRECTION('',(1.,0.,0.));
#11212=DIRECTION('',(0.,1.,0.));
#11213=DIRECTION('',(-1.,0.,0.));
#11214=DIRECTION('center_axis',(0.,0.,-1.));
#11215=DIRECTION('ref_axis',(1.,0.,0.));
#11216=DIRECTION('center_axis',(0.,0.,-1.));
#11217=DIRECTION('ref_axis',(1.,0.,0.));
#11218=DIRECTION('',(0.,-1.,0.));
#11219=DIRECTION('',(-1.,0.,0.));
#11220=DIRECTION('',(0.,1.,0.));
#11221=DIRECTION('',(0.,1.,0.));
#11222=DIRECTION('',(1.,0.,0.));
#11223=DIRECTION('',(0.,-1.,0.));
#11224=DIRECTION('center_axis',(0.,1.,0.));
#11225=DIRECTION('ref_axis',(6.12323399573677E-17,0.,1.));
#11226=DIRECTION('center_axis',(0.,1.,0.));
#11227=DIRECTION('ref_axis',(1.,0.,0.));
#11228=DIRECTION('center_axis',(0.,-1.,0.));
#11229=DIRECTION('ref_axis',(1.,0.,0.));
#11230=DIRECTION('center_axis',(0.,1.,0.));
#11231=DIRECTION('ref_axis',(1.,0.,0.));
#11232=DIRECTION('center_axis',(0.,1.,0.));
#11233=DIRECTION('ref_axis',(1.,0.,0.));
#11234=DIRECTION('center_axis',(0.,1.,0.));
#11235=DIRECTION('ref_axis',(-1.,0.,0.));
#11236=DIRECTION('',(-1.,0.,0.));
#11237=DIRECTION('',(0.,0.,1.));
#11238=DIRECTION('',(-1.,0.,0.));
#11239=DIRECTION('',(0.,0.,1.));
#11240=DIRECTION('center_axis',(1.,0.,0.));
#11241=DIRECTION('ref_axis',(0.,1.,0.));
#11242=DIRECTION('',(0.,1.,0.));
#11243=DIRECTION('',(0.,0.,1.));
#11244=DIRECTION('',(0.,1.,0.));
#11245=DIRECTION('center_axis',(0.,-1.,0.));
#11246=DIRECTION('ref_axis',(1.,0.,0.));
#11247=DIRECTION('',(1.,0.,0.));
#11248=DIRECTION('',(0.,0.,1.));
#11249=DIRECTION('',(1.,0.,0.));
#11250=DIRECTION('center_axis',(-1.,0.,0.));
#11251=DIRECTION('ref_axis',(0.,-1.,0.));
#11252=DIRECTION('',(0.,-1.,0.));
#11253=DIRECTION('',(0.,-1.,0.));
#11254=DIRECTION('center_axis',(0.,0.,1.));
#11255=DIRECTION('ref_axis',(1.,0.,0.));
#11256=DIRECTION('center_axis',(0.,0.,1.));
#11257=DIRECTION('ref_axis',(1.,0.,0.));
#11258=DIRECTION('center_axis',(0.,0.,1.));
#11259=DIRECTION('ref_axis',(1.,0.,0.));
#11260=DIRECTION('',(0.,0.,1.));
#11261=DIRECTION('center_axis',(0.,0.,1.));
#11262=DIRECTION('ref_axis',(1.,0.,0.));
#11263=DIRECTION('center_axis',(0.,0.,1.));
#11264=DIRECTION('ref_axis',(1.,0.,0.));
#11265=DIRECTION('',(0.,0.,1.));
#11266=DIRECTION('center_axis',(0.,1.,0.));
#11267=DIRECTION('ref_axis',(-1.,0.,0.));
#11268=DIRECTION('',(-1.,0.,0.));
#11269=DIRECTION('',(0.,0.,1.));
#11270=DIRECTION('',(0.,0.,1.));
#11271=DIRECTION('center_axis',(1.,0.,0.));
#11272=DIRECTION('ref_axis',(0.,1.,0.));
#11273=DIRECTION('',(0.,1.,0.));
#11274=DIRECTION('',(0.,0.,1.));
#11275=DIRECTION('center_axis',(0.,-1.,0.));
#11276=DIRECTION('ref_axis',(1.,0.,0.));
#11277=DIRECTION('',(1.,0.,0.));
#11278=DIRECTION('',(0.,0.,1.));
#11279=DIRECTION('center_axis',(-1.,0.,0.));
#11280=DIRECTION('ref_axis',(0.,-1.,0.));
#11281=DIRECTION('',(0.,-1.,0.));
#11282=DIRECTION('center_axis',(0.,0.,1.));
#11283=DIRECTION('ref_axis',(1.,0.,0.));
#13867=CARTESIAN_POINT('',(0.,0.,0.));
#13868=CARTESIAN_POINT('Origin',(0.,0.,0.));
#13869=CARTESIAN_POINT('',(-2.05,-1.65,2.51052593825207E-16));
#13870=CARTESIAN_POINT('Origin',(0.,-1.65,0.));
#13871=CARTESIAN_POINT('',(-2.05,-1.14891252930761,-2.51052593825207E-16));
#13872=CARTESIAN_POINT('',(-2.05,0.,2.51052593825207E-16));
#13873=CARTESIAN_POINT('Origin',(0.,-1.14891252930761,0.));
#13874=CARTESIAN_POINT('Origin',(0.,0.,0.));
#13875=CARTESIAN_POINT('',(-2.05,1.14891252930761,2.51052593825207E-16));
#13876=CARTESIAN_POINT('Origin',(0.,1.14891252930761,0.));
#13877=CARTESIAN_POINT('',(-2.05,1.65,-2.51052593825207E-16));
#13878=CARTESIAN_POINT('',(-2.05,0.,2.51052593825207E-16));
#13879=CARTESIAN_POINT('Origin',(0.,1.65,0.));
#13880=CARTESIAN_POINT('Origin',(0.,0.,0.));
#13881=CARTESIAN_POINT('',(-1.43895998899814E-16,-1.76221774462768E-32,
-2.35));
#13882=CARTESIAN_POINT('',(-1.43895998899814E-16,-1.76221774462768E-32,
2.35));
#13883=CARTESIAN_POINT('Origin',(0.,0.,0.));
#13884=CARTESIAN_POINT('Origin',(0.,1.55,-1.49));
#13885=CARTESIAN_POINT('',(-3.76384615384615,1.55,-2.13));
#13886=CARTESIAN_POINT('',(-1.81744325908679,1.55,-2.13));
#13887=CARTESIAN_POINT('',(0.,1.55,-2.13));
#13888=CARTESIAN_POINT('',(-2.46585583768694,1.55,-1.32648218523477));
#13889=CARTESIAN_POINT('',(-1.68,1.55,-0.84));
#13890=CARTESIAN_POINT('Origin',(0.,1.55,0.));
#13891=CARTESIAN_POINT('Origin',(0.,1.55,-1.49));
#13892=CARTESIAN_POINT('',(1.81744325908679,1.55,-2.13));
#13893=CARTESIAN_POINT('',(3.76384615384615,1.55,-2.13));
#13894=CARTESIAN_POINT('',(0.,1.55,-2.13));
#13895=CARTESIAN_POINT('',(2.46585583768694,1.55,-1.32648218523477));
#13896=CARTESIAN_POINT('Origin',(0.,1.55,0.));
#13897=CARTESIAN_POINT('',(3.78,1.55,-2.14));
#13898=CARTESIAN_POINT('Origin',(0.,-1.55,-1.49));
#13899=CARTESIAN_POINT('',(-1.81744325908679,-1.55,-2.13));
#13900=CARTESIAN_POINT('',(-3.76384615384615,-1.55,-2.13));
#13901=CARTESIAN_POINT('',(0.,-1.55,-2.13));
#13902=CARTESIAN_POINT('',(-2.46585583768694,-1.55,-1.32648218523477));
#13903=CARTESIAN_POINT('Origin',(0.,-1.55,0.));
#13904=CARTESIAN_POINT('',(-1.68,-1.55,-0.84));
#13905=CARTESIAN_POINT('Origin',(-3.78,0.,-2.14));
#13906=CARTESIAN_POINT('',(-3.76384615384615,0.,-2.13));
#13907=CARTESIAN_POINT('',(-2.46585583768694,0.,-1.32648218523477));
#13908=CARTESIAN_POINT('Origin',(0.,-1.55,-1.49));
#13909=CARTESIAN_POINT('',(3.76384615384615,-1.55,-2.13));
#13910=CARTESIAN_POINT('',(1.81744325908679,-1.55,-2.13));
#13911=CARTESIAN_POINT('',(0.,-1.55,-2.13));
#13912=CARTESIAN_POINT('',(2.46585583768694,-1.55,-1.32648218523477));
#13913=CARTESIAN_POINT('',(3.78,-1.55,-2.14));
#13914=CARTESIAN_POINT('Origin',(0.,-1.55,0.));
#13915=CARTESIAN_POINT('Origin',(1.68,0.,-0.84));
#13916=CARTESIAN_POINT('',(3.76384615384615,0.,-2.13));
#13917=CARTESIAN_POINT('',(2.46585583768694,0.,-1.32648218523477));
#13918=CARTESIAN_POINT('Origin',(0.,0.,-2.13));
#13919=CARTESIAN_POINT('',(-6.35,1.9,-2.13));
#13920=CARTESIAN_POINT('',(-6.35,-1.9,-2.13));
#13921=CARTESIAN_POINT('',(-6.35,1.9,-2.13));
#13922=CARTESIAN_POINT('',(6.35,-1.9,-2.13));
#13923=CARTESIAN_POINT('',(-6.35,-1.9,-2.13));
#13924=CARTESIAN_POINT('',(6.35,1.9,-2.13));
#13925=CARTESIAN_POINT('',(6.35,-1.9,-2.13));
#13926=CARTESIAN_POINT('',(6.35,1.9,-2.13));
#13927=CARTESIAN_POINT('',(4.1,7.9602041944578E-17,-2.13));
#13928=CARTESIAN_POINT('Origin',(4.75,0.,-2.13));
#13929=CARTESIAN_POINT('',(-5.4,7.9602041944578E-17,-2.13));
#13930=CARTESIAN_POINT('Origin',(-4.75,0.,-2.13));
#13931=CARTESIAN_POINT('',(1.81744325908679,-1.65,-2.13));
#13932=CARTESIAN_POINT('',(1.81744325908679,0.,-2.13));
#13933=CARTESIAN_POINT('',(-1.81744325908679,-1.65,-2.13));
#13934=CARTESIAN_POINT('',(0.,-1.65,-2.13));
#13935=CARTESIAN_POINT('',(-1.81744325908679,0.,-2.13));
#13936=CARTESIAN_POINT('',(-1.81744325908679,1.65,-2.13));
#13937=CARTESIAN_POINT('',(-1.81744325908679,0.,-2.13));
#13938=CARTESIAN_POINT('',(1.81744325908679,1.65,-2.13));
#13939=CARTESIAN_POINT('',(0.,1.65,-2.13));
#13940=CARTESIAN_POINT('',(1.81744325908679,0.,-2.13));
#13941=CARTESIAN_POINT('Origin',(0.,0.,0.));
#13942=CARTESIAN_POINT('Origin',(0.,1.65,0.));
#13943=CARTESIAN_POINT('Origin',(0.,-1.65,0.));
#13944=CARTESIAN_POINT('Origin',(0.,-1.65,0.));
#13945=CARTESIAN_POINT('Origin',(0.,1.65,0.));
#13946=CARTESIAN_POINT('Origin',(3.35,1.4,-3.33));
#13947=CARTESIAN_POINT('',(3.35,1.4,-3.33));
#13948=CARTESIAN_POINT('',(-3.35,1.4,-3.33));
#13949=CARTESIAN_POINT('',(1.675,1.4,-3.33));
#13950=CARTESIAN_POINT('',(3.35,1.4,-2.83));
#13951=CARTESIAN_POINT('',(3.35,1.4,-3.33));
#13952=CARTESIAN_POINT('',(-3.35,1.4,-2.83));
#13953=CARTESIAN_POINT('',(3.35,1.4,-2.83));
#13954=CARTESIAN_POINT('',(-3.35,1.4,-3.33));
#13955=CARTESIAN_POINT('Origin',(3.35,-1.4,-3.33));
#13956=CARTESIAN_POINT('',(3.35,-1.4,-3.33));
#13957=CARTESIAN_POINT('',(3.35,-0.7,-3.33));
#13958=CARTESIAN_POINT('',(3.35,-1.4,-2.83));
#13959=CARTESIAN_POINT('',(3.35,-1.4,-3.33));
#13960=CARTESIAN_POINT('',(3.35,-1.4,-2.83));
#13961=CARTESIAN_POINT('Origin',(-3.35,-1.4,-3.33));
#13962=CARTESIAN_POINT('',(-3.35,-1.4,-3.33));
#13963=CARTESIAN_POINT('',(-1.675,-1.4,-3.33));
#13964=CARTESIAN_POINT('',(-3.35,-1.4,-2.83));
#13965=CARTESIAN_POINT('',(-3.35,-1.4,-3.33));
#13966=CARTESIAN_POINT('',(-3.35,-1.4,-2.83));
#13967=CARTESIAN_POINT('Origin',(-3.35,1.4,-3.33));
#13968=CARTESIAN_POINT('',(-3.35,0.7,-3.33));
#13969=CARTESIAN_POINT('',(-3.35,1.4,-2.83));
#13970=CARTESIAN_POINT('Origin',(0.,0.,-2.83));
#13971=CARTESIAN_POINT('Origin',(-4.75,0.,-3.33));
#13972=CARTESIAN_POINT('',(-5.4,-7.9602041944578E-17,-3.33));
#13973=CARTESIAN_POINT('Origin',(-4.75,0.,-3.33));
#13974=CARTESIAN_POINT('',(-5.4,-7.9602041944578E-17,-3.33));
#13975=CARTESIAN_POINT('Origin',(4.75,0.,-3.33));
#13976=CARTESIAN_POINT('',(4.1,-7.9602041944578E-17,-3.33));
#13977=CARTESIAN_POINT('Origin',(4.75,0.,-3.33));
#13978=CARTESIAN_POINT('',(4.1,-7.9602041944578E-17,-3.33));
#13979=CARTESIAN_POINT('Origin',(6.35,1.9,-3.33));
#13980=CARTESIAN_POINT('',(6.35,1.9,-3.33));
#13981=CARTESIAN_POINT('',(-6.35,1.9,-3.33));
#13982=CARTESIAN_POINT('',(6.35,1.9,-3.33));
#13983=CARTESIAN_POINT('',(-6.35,1.9,-3.33));
#13984=CARTESIAN_POINT('',(6.35,1.9,-3.33));
#13985=CARTESIAN_POINT('Origin',(6.35,-1.9,-3.33));
#13986=CARTESIAN_POINT('',(6.35,-1.9,-3.33));
#13987=CARTESIAN_POINT('',(6.35,-1.9,-3.33));
#13988=CARTESIAN_POINT('',(6.35,-1.9,-3.33));
#13989=CARTESIAN_POINT('Origin',(-6.35,-1.9,-3.33));
#13990=CARTESIAN_POINT('',(-6.35,-1.9,-3.33));
#13991=CARTESIAN_POINT('',(-6.35,-1.9,-3.33));
#13992=CARTESIAN_POINT('',(-6.35,-1.9,-3.33));
#13993=CARTESIAN_POINT('Origin',(-6.35,1.9,-3.33));
#13994=CARTESIAN_POINT('',(-6.35,1.9,-3.33));
#13995=CARTESIAN_POINT('Origin',(0.,0.,-3.33));
#16807=UNCERTAINTY_MEASURE_WITH_UNIT(LENGTH_MEASURE(0.001),#16912,
'DISTANCE_ACCURACY_VALUE',
'Maximum model space distance between geometric entities at asserted c
onnectivities');
#16852=UNCERTAINTY_MEASURE_WITH_UNIT(LENGTH_MEASURE(0.001),#16912,
'DISTANCE_ACCURACY_VALUE',
'Maximum model space distance between geometric entities at asserted c
onnectivities');
#16866=(
GEOMETRIC_REPRESENTATION_CONTEXT(3)
GLOBAL_UNCERTAINTY_ASSIGNED_CONTEXT((#16807))
GLOBAL_UNIT_ASSIGNED_CONTEXT((#16912,#16914,#16915))
REPRESENTATION_CONTEXT('','3D')
);
#16911=(
GEOMETRIC_REPRESENTATION_CONTEXT(3)
GLOBAL_UNCERTAINTY_ASSIGNED_CONTEXT((#16852))
GLOBAL_UNIT_ASSIGNED_CONTEXT((#16912,#16914,#16915))
REPRESENTATION_CONTEXT('','3D')
);
#16912=(
LENGTH_UNIT()
NAMED_UNIT(*)
SI_UNIT(.CENTI.,.METRE.)
);
#16914=(
NAMED_UNIT(*)
PLANE_ANGLE_UNIT()
SI_UNIT($,.RADIAN.)
);
#16915=(
NAMED_UNIT(*)
SI_UNIT($,.STERADIAN.)
SOLID_ANGLE_UNIT()
);
#16929=SHAPE_DEFINITION_REPRESENTATION(#16987,#17137);
#16987=PRODUCT_DEFINITION_SHAPE('',$,#17196);
#17137=SHAPE_REPRESENTATION('',(#9726),#16866);
#17182=PRODUCT_DEFINITION_CONTEXT('part definition',#17358,'design');
#17196=PRODUCT_DEFINITION('Housing','Housing',#17254,#17182);
#17254=PRODUCT_DEFINITION_FORMATION('',$,#17373);
#17358=APPLICATION_CONTEXT(
'Core Data for Automotive Mechanical Design Process');
#17359=PRODUCT_CONTEXT('part definition',#17358,'mechanical');
#17373=PRODUCT('Housing','Housing','Housing',(#17359));
#17460=COLOUR_RGB('Dark Blue',0.08,0.2,0.34);
#17461=FILL_AREA_STYLE_COLOUR('',#17460);
#17462=FILL_AREA_STYLE('',(#17461));
#17463=SURFACE_STYLE_FILL_AREA(#17462);
#17464=SURFACE_SIDE_STYLE('',(#17463));
#17465=SURFACE_STYLE_USAGE(.BOTH.,#17464);
#17466=PRESENTATION_STYLE_ASSIGNMENT((#17465));
ENDSEC;
END-ISO-10303-21;
